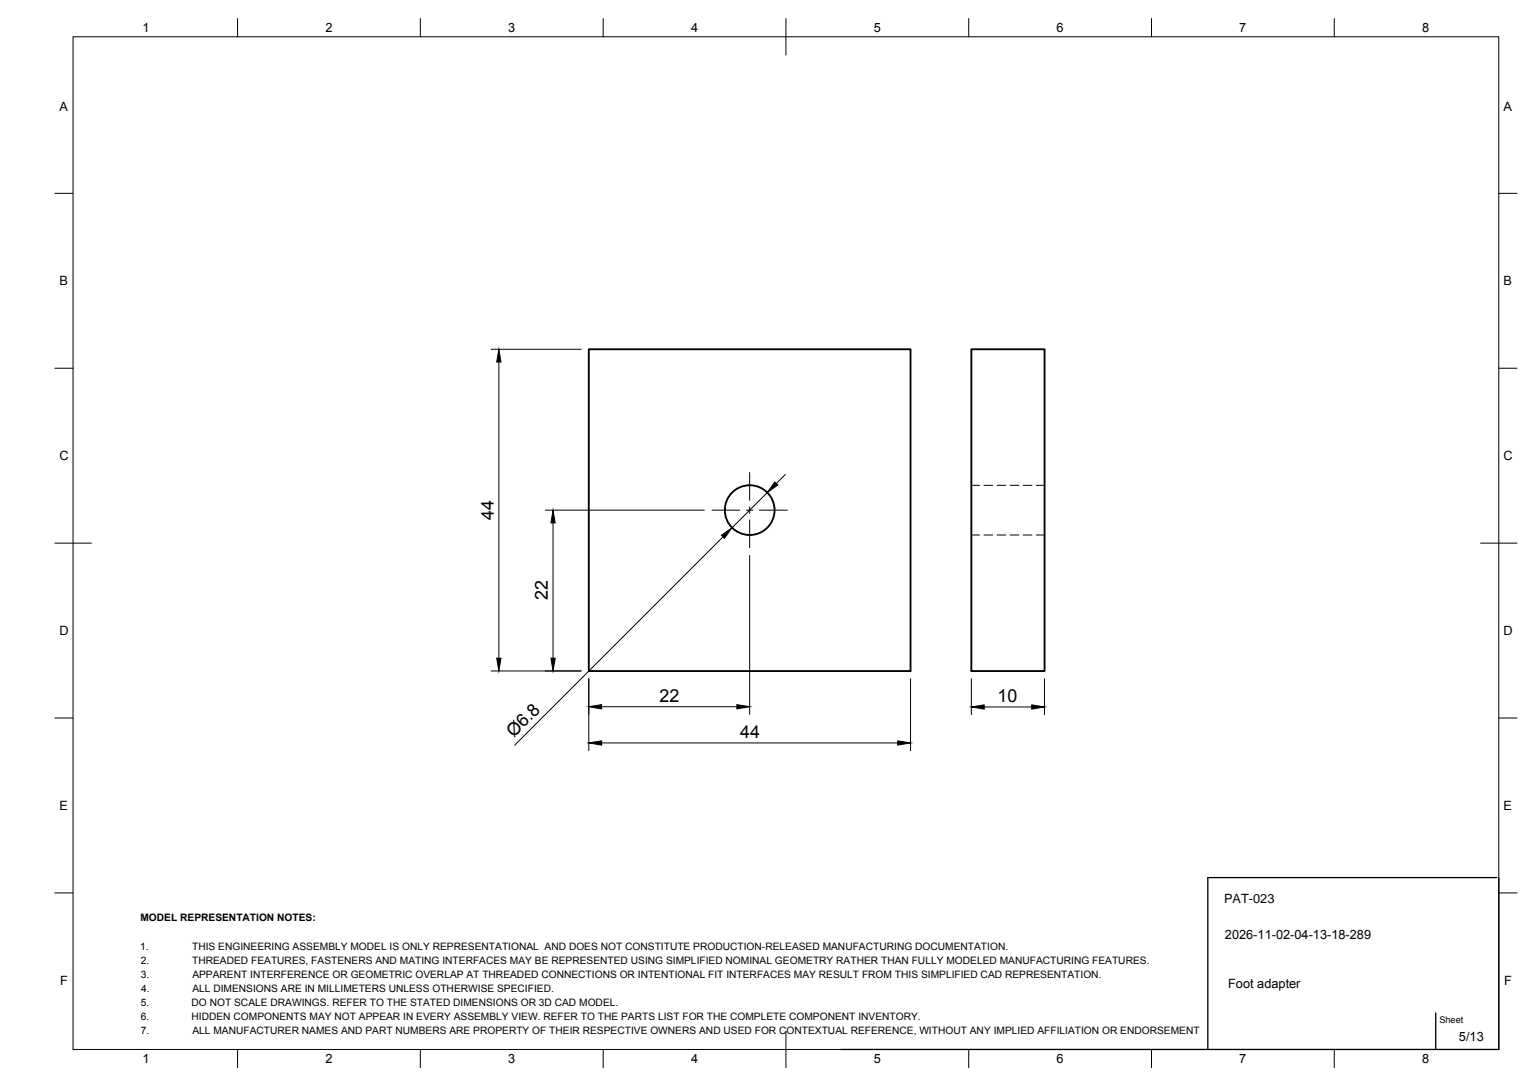
ISO-10303-21;
HEADER;
/* Generated by software containing ST-Developer
 * from STEP Tools, Inc. (www.steptools.com) 
 */

FILE_DESCRIPTION(
/* description */ ('PAT-023'),
/* implementation_level */ '2;1');

FILE_NAME(
/* name */ 'Foot adapter.step',
/* time_stamp */ '2026-10-29T15:47:46-07:00',
/* author */ (''),
/* organization */ (''),
/* preprocessor_version */ 'ST-DEVELOPER v20.2',
/* originating_system */ 'Autodesk Translation Framework v15.17.0.0',
/* authorisation */ '');

FILE_SCHEMA (('AUTOMOTIVE_DESIGN { 1 0 10303 214 3 1 1 }'));
ENDSEC;

DATA;
#10=MECHANICAL_DESIGN_GEOMETRIC_PRESENTATION_REPRESENTATION('',(#84),#3773);
#68=SHAPE_REPRESENTATION_RELATIONSHIP('SRR','None',#3815,#76);
#76=ADVANCED_BREP_SHAPE_REPRESENTATION('',(#92),#3763);
#84=STYLED_ITEM('',(#3960),#92);
#92=MANIFOLD_SOLID_BREP('Body1',#2237);
#100=FACE_BOUND('',#343,.T.);
#101=FACE_BOUND('',#345,.T.);
#115=PLANE('',#2340);
#116=PLANE('',#2341);
#117=PLANE('',#2342);
#118=PLANE('',#2343);
#119=PLANE('',#2344);
#120=PLANE('',#2345);
#218=FACE_OUTER_BOUND('',#337,.T.);
#219=FACE_OUTER_BOUND('',#338,.T.);
#220=FACE_OUTER_BOUND('',#339,.T.);
#221=FACE_OUTER_BOUND('',#340,.T.);
#222=FACE_OUTER_BOUND('',#341,.T.);
#223=FACE_OUTER_BOUND('',#342,.T.);
#224=FACE_OUTER_BOUND('',#344,.T.);
#337=EDGE_LOOP('',(#1517,#1518,#1519,#1520));
#338=EDGE_LOOP('',(#1521,#1522,#1523,#1524));
#339=EDGE_LOOP('',(#1525,#1526,#1527,#1528));
#340=EDGE_LOOP('',(#1529,#1530,#1531,#1532));
#341=EDGE_LOOP('',(#1533,#1534,#1535,#1536));
#342=EDGE_LOOP('',(#1537,#1538,#1539,#1540));
#343=EDGE_LOOP('',(#1541));
#344=EDGE_LOOP('',(#1542,#1543,#1544,#1545));
#345=EDGE_LOOP('',(#1546));
#471=LINE('',#3109,#735);
#472=LINE('',#3114,#736);
#473=LINE('',#3116,#737);
#474=LINE('',#3118,#738);
#475=LINE('',#3119,#739);
#476=LINE('',#3122,#740);
#477=LINE('',#3124,#741);
#478=LINE('',#3125,#742);
#479=LINE('',#3128,#743);
#480=LINE('',#3130,#744);
#481=LINE('',#3131,#745);
#482=LINE('',#3133,#746);
#483=LINE('',#3134,#747);
#735=VECTOR('',#2512,0.34);
#736=VECTOR('',#2517,1.);
#737=VECTOR('',#2518,1.);
#738=VECTOR('',#2519,1.);
#739=VECTOR('',#2520,1.);
#740=VECTOR('',#2523,1.);
#741=VECTOR('',#2524,1.);
#742=VECTOR('',#2525,1.);
#743=VECTOR('',#2528,1.);
#744=VECTOR('',#2529,1.);
#745=VECTOR('',#2530,1.);
#746=VECTOR('',#2533,1.);
#747=VECTOR('',#2534,1.);
#999=CIRCLE('',#2338,0.34);
#1000=CIRCLE('',#2339,0.34);
#1025=VERTEX_POINT('',#3106);
#1026=VERTEX_POINT('',#3108);
#1027=VERTEX_POINT('',#3112);
#1028=VERTEX_POINT('',#3113);
#1029=VERTEX_POINT('',#3115);
#1030=VERTEX_POINT('',#3117);
#1031=VERTEX_POINT('',#3121);
#1032=VERTEX_POINT('',#3123);
#1033=VERTEX_POINT('',#3127);
#1034=VERTEX_POINT('',#3129);
#1221=EDGE_CURVE('',#1025,#1025,#999,.T.);
#1222=EDGE_CURVE('',#1025,#1026,#471,.T.);
#1223=EDGE_CURVE('',#1026,#1026,#1000,.T.);
#1224=EDGE_CURVE('',#1027,#1028,#472,.T.);
#1225=EDGE_CURVE('',#1028,#1029,#473,.T.);
#1226=EDGE_CURVE('',#1030,#1029,#474,.T.);
#1227=EDGE_CURVE('',#1027,#1030,#475,.T.);
#1228=EDGE_CURVE('',#1031,#1027,#476,.T.);
#1229=EDGE_CURVE('',#1032,#1030,#477,.T.);
#1230=EDGE_CURVE('',#1031,#1032,#478,.T.);
#1231=EDGE_CURVE('',#1033,#1031,#479,.T.);
#1232=EDGE_CURVE('',#1034,#1032,#480,.T.);
#1233=EDGE_CURVE('',#1033,#1034,#481,.T.);
#1234=EDGE_CURVE('',#1028,#1033,#482,.T.);
#1235=EDGE_CURVE('',#1029,#1034,#483,.T.);
#1517=ORIENTED_EDGE('',*,*,#1221,.F.);
#1518=ORIENTED_EDGE('',*,*,#1222,.T.);
#1519=ORIENTED_EDGE('',*,*,#1223,.F.);
#1520=ORIENTED_EDGE('',*,*,#1222,.F.);
#1521=ORIENTED_EDGE('',*,*,#1224,.T.);
#1522=ORIENTED_EDGE('',*,*,#1225,.T.);
#1523=ORIENTED_EDGE('',*,*,#1226,.F.);
#1524=ORIENTED_EDGE('',*,*,#1227,.F.);
#1525=ORIENTED_EDGE('',*,*,#1228,.T.);
#1526=ORIENTED_EDGE('',*,*,#1227,.T.);
#1527=ORIENTED_EDGE('',*,*,#1229,.F.);
#1528=ORIENTED_EDGE('',*,*,#1230,.F.);
#1529=ORIENTED_EDGE('',*,*,#1231,.T.);
#1530=ORIENTED_EDGE('',*,*,#1230,.T.);
#1531=ORIENTED_EDGE('',*,*,#1232,.F.);
#1532=ORIENTED_EDGE('',*,*,#1233,.F.);
#1533=ORIENTED_EDGE('',*,*,#1234,.T.);
#1534=ORIENTED_EDGE('',*,*,#1233,.T.);
#1535=ORIENTED_EDGE('',*,*,#1235,.F.);
#1536=ORIENTED_EDGE('',*,*,#1225,.F.);
#1537=ORIENTED_EDGE('',*,*,#1235,.T.);
#1538=ORIENTED_EDGE('',*,*,#1232,.T.);
#1539=ORIENTED_EDGE('',*,*,#1229,.T.);
#1540=ORIENTED_EDGE('',*,*,#1226,.T.);
#1541=ORIENTED_EDGE('',*,*,#1223,.T.);
#1542=ORIENTED_EDGE('',*,*,#1234,.F.);
#1543=ORIENTED_EDGE('',*,*,#1224,.F.);
#1544=ORIENTED_EDGE('',*,*,#1228,.F.);
#1545=ORIENTED_EDGE('',*,*,#1231,.F.);
#1546=ORIENTED_EDGE('',*,*,#1221,.T.);
#2109=CYLINDRICAL_SURFACE('',#2337,0.34);
#2118=ADVANCED_FACE('',(#218),#2109,.F.);
#2119=ADVANCED_FACE('',(#219),#115,.T.);
#2120=ADVANCED_FACE('',(#220),#116,.T.);
#2121=ADVANCED_FACE('',(#221),#117,.T.);
#2122=ADVANCED_FACE('',(#222),#118,.T.);
#2123=ADVANCED_FACE('',(#223,#100),#119,.T.);
#2124=ADVANCED_FACE('',(#224,#101),#120,.F.);
#2237=CLOSED_SHELL('',(#2118,#2119,#2120,#2121,#2122,#2123,#2124));
#2336=AXIS2_PLACEMENT_3D('',#3104,#2506,#2507);
#2337=AXIS2_PLACEMENT_3D('',#3105,#2508,#2509);
#2338=AXIS2_PLACEMENT_3D('',#3107,#2510,#2511);
#2339=AXIS2_PLACEMENT_3D('',#3110,#2513,#2514);
#2340=AXIS2_PLACEMENT_3D('',#3111,#2515,#2516);
#2341=AXIS2_PLACEMENT_3D('',#3120,#2521,#2522);
#2342=AXIS2_PLACEMENT_3D('',#3126,#2526,#2527);
#2343=AXIS2_PLACEMENT_3D('',#3132,#2531,#2532);
#2344=AXIS2_PLACEMENT_3D('',#3135,#2535,#2536);
#2345=AXIS2_PLACEMENT_3D('',#3136,#2537,#2538);
#2506=DIRECTION('axis',(0.,0.,1.));
#2507=DIRECTION('refdir',(1.,0.,0.));
#2508=DIRECTION('center_axis',(0.,0.,1.));
#2509=DIRECTION('ref_axis',(1.,0.,0.));
#2510=DIRECTION('center_axis',(0.,0.,1.));
#2511=DIRECTION('ref_axis',(1.,0.,0.));
#2512=DIRECTION('',(0.,0.,1.));
#2513=DIRECTION('center_axis',(0.,0.,-1.));
#2514=DIRECTION('ref_axis',(1.,0.,0.));
#2515=DIRECTION('center_axis',(0.,1.,0.));
#2516=DIRECTION('ref_axis',(-1.,0.,0.));
#2517=DIRECTION('',(-1.,0.,0.));
#2518=DIRECTION('',(0.,0.,1.));
#2519=DIRECTION('',(-1.,0.,0.));
#2520=DIRECTION('',(0.,0.,1.));
#2521=DIRECTION('center_axis',(1.,0.,0.));
#2522=DIRECTION('ref_axis',(0.,1.,0.));
#2523=DIRECTION('',(0.,1.,0.));
#2524=DIRECTION('',(0.,1.,0.));
#2525=DIRECTION('',(0.,0.,1.));
#2526=DIRECTION('center_axis',(0.,-1.,0.));
#2527=DIRECTION('ref_axis',(1.,0.,0.));
#2528=DIRECTION('',(1.,0.,0.));
#2529=DIRECTION('',(1.,0.,0.));
#2530=DIRECTION('',(0.,0.,1.));
#2531=DIRECTION('center_axis',(-1.,0.,0.));
#2532=DIRECTION('ref_axis',(0.,-1.,0.));
#2533=DIRECTION('',(0.,-1.,0.));
#2534=DIRECTION('',(0.,-1.,0.));
#2535=DIRECTION('center_axis',(0.,0.,1.));
#2536=DIRECTION('ref_axis',(1.,0.,0.));
#2537=DIRECTION('center_axis',(0.,0.,1.));
#2538=DIRECTION('ref_axis',(1.,0.,0.));
#3104=CARTESIAN_POINT('',(0.,0.,0.));
#3105=CARTESIAN_POINT('Origin',(0.,0.,5.9));
#3106=CARTESIAN_POINT('',(-0.34,-4.163799117101E-17,6.));
#3107=CARTESIAN_POINT('Origin',(0.,0.,6.));
#3108=CARTESIAN_POINT('',(-0.34,4.163799117101E-17,7.));
#3109=CARTESIAN_POINT('',(-0.34,-4.163799117101E-17,5.9));
#3110=CARTESIAN_POINT('Origin',(0.,0.,7.));
#3111=CARTESIAN_POINT('Origin',(2.2,2.2,6.));
#3112=CARTESIAN_POINT('',(2.2,2.2,6.));
#3113=CARTESIAN_POINT('',(-2.2,2.2,6.));
#3114=CARTESIAN_POINT('',(2.2,2.2,6.));
#3115=CARTESIAN_POINT('',(-2.2,2.2,7.));
#3116=CARTESIAN_POINT('',(-2.2,2.2,6.));
#3117=CARTESIAN_POINT('',(2.2,2.2,7.));
#3118=CARTESIAN_POINT('',(2.2,2.2,7.));
#3119=CARTESIAN_POINT('',(2.2,2.2,6.));
#3120=CARTESIAN_POINT('Origin',(2.2,-2.2,6.));
#3121=CARTESIAN_POINT('',(2.2,-2.2,6.));
#3122=CARTESIAN_POINT('',(2.2,-2.2,6.));
#3123=CARTESIAN_POINT('',(2.2,-2.2,7.));
#3124=CARTESIAN_POINT('',(2.2,-2.2,7.));
#3125=CARTESIAN_POINT('',(2.2,-2.2,6.));
#3126=CARTESIAN_POINT('Origin',(-2.2,-2.2,6.));
#3127=CARTESIAN_POINT('',(-2.2,-2.2,6.));
#3128=CARTESIAN_POINT('',(-2.2,-2.2,6.));
#3129=CARTESIAN_POINT('',(-2.2,-2.2,7.));
#3130=CARTESIAN_POINT('',(-2.2,-2.2,7.));
#3131=CARTESIAN_POINT('',(-2.2,-2.2,6.));
#3132=CARTESIAN_POINT('Origin',(-2.2,2.2,6.));
#3133=CARTESIAN_POINT('',(-2.2,2.2,6.));
#3134=CARTESIAN_POINT('',(-2.2,2.2,7.));
#3135=CARTESIAN_POINT('Origin',(0.,0.,7.));
#3136=CARTESIAN_POINT('Origin',(0.,0.,6.));
#3750=UNCERTAINTY_MEASURE_WITH_UNIT(LENGTH_MEASURE(0.001),#3774,
'DISTANCE_ACCURACY_VALUE',
'Maximum model space distance between geometric entities at asserted c
onnectivities');
#3760=UNCERTAINTY_MEASURE_WITH_UNIT(LENGTH_MEASURE(0.001),#3774,
'DISTANCE_ACCURACY_VALUE',
'Maximum model space distance between geometric entities at asserted c
onnectivities');
#3763=(
GEOMETRIC_REPRESENTATION_CONTEXT(3)
GLOBAL_UNCERTAINTY_ASSIGNED_CONTEXT((#3750))
GLOBAL_UNIT_ASSIGNED_CONTEXT((#3774,#3776,#3777))
REPRESENTATION_CONTEXT('','3D')
);
#3773=(
GEOMETRIC_REPRESENTATION_CONTEXT(3)
GLOBAL_UNCERTAINTY_ASSIGNED_CONTEXT((#3760))
GLOBAL_UNIT_ASSIGNED_CONTEXT((#3774,#3776,#3777))
REPRESENTATION_CONTEXT('','3D')
);
#3774=(
LENGTH_UNIT()
NAMED_UNIT(*)
SI_UNIT(.CENTI.,.METRE.)
);
#3776=(
NAMED_UNIT(*)
PLANE_ANGLE_UNIT()
SI_UNIT($,.RADIAN.)
);
#3777=(
NAMED_UNIT(*)
SI_UNIT($,.STERADIAN.)
SOLID_ANGLE_UNIT()
);
#3780=SHAPE_DEFINITION_REPRESENTATION(#3792,#3815);
#3792=PRODUCT_DEFINITION_SHAPE('',$,#3828);
#3815=SHAPE_REPRESENTATION('',(#2336),#3763);
#3825=PRODUCT_DEFINITION_CONTEXT('part definition',#3863,'design');
#3828=PRODUCT_DEFINITION('Foot adapter','Foot adapter',#3840,
#3825);
#3840=PRODUCT_DEFINITION_FORMATION('',$,#3867);
#3863=APPLICATION_CONTEXT(
'Core Data for Automotive Mechanical Design Process');
#3864=PRODUCT_CONTEXT('part definition',#3863,'mechanical');
#3867=PRODUCT('Foot adapter','Foot adapter','Foot adapter',(#3864));
#3954=COLOUR_RGB('Off White',0.89,0.88,0.83);
#3955=FILL_AREA_STYLE_COLOUR('',#3954);
#3956=FILL_AREA_STYLE('',(#3955));
#3957=SURFACE_STYLE_FILL_AREA(#3956);
#3958=SURFACE_SIDE_STYLE('',(#3957));
#3959=SURFACE_STYLE_USAGE(.BOTH.,#3958);
#3960=PRESENTATION_STYLE_ASSIGNMENT((#3959));
ENDSEC;
END-ISO-10303-21;
